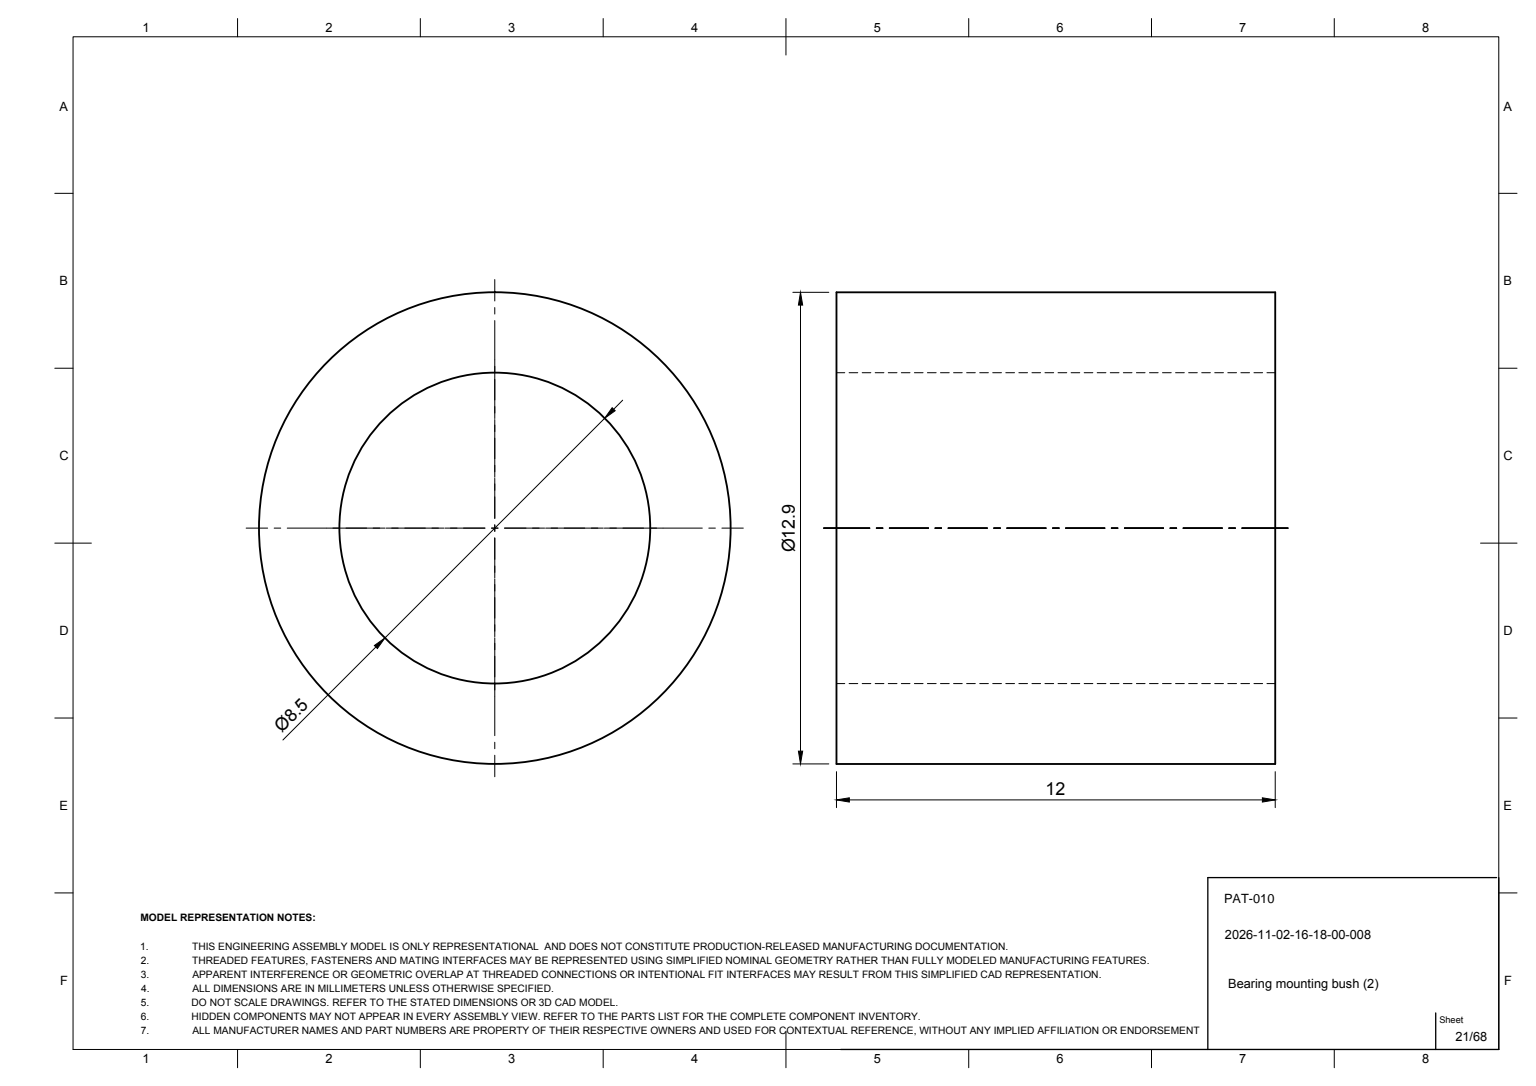
ISO-10303-21;
HEADER;
/* Generated by software containing ST-Developer
 * from STEP Tools, Inc. (www.steptools.com) 
 */

FILE_DESCRIPTION(
/* description */ ('Belt conveyor head drive unit'),
/* implementation_level */ '2;1');

FILE_NAME(
/* name */ 'Bearing mounting bush (2).step',
/* time_stamp */ '2026-10-28T03:26:19-07:00',
/* author */ (''),
/* organization */ (''),
/* preprocessor_version */ 'ST-DEVELOPER v20.2',
/* originating_system */ 'Autodesk Translation Framework v15.17.0.0',
/* authorisation */ '');

FILE_SCHEMA (('AUTOMOTIVE_DESIGN { 1 0 10303 214 3 1 1 }'));
ENDSEC;

DATA;
#10=MECHANICAL_DESIGN_GEOMETRIC_PRESENTATION_REPRESENTATION('',(#867),#27069);
#729=SHAPE_REPRESENTATION_RELATIONSHIP('SRR','None',#27373,#798);
#798=ADVANCED_BREP_SHAPE_REPRESENTATION('',(#952),#27015);
#867=STYLED_ITEM('',(#27797),#952);
#952=MANIFOLD_SOLID_BREP('Body1',#13732);
#1125=FACE_BOUND('',#2799,.T.);
#1126=FACE_BOUND('',#2801,.T.);
#1401=PLANE('',#15105);
#1402=PLANE('',#15106);
#1883=FACE_OUTER_BOUND('',#2796,.T.);
#1884=FACE_OUTER_BOUND('',#2797,.T.);
#1885=FACE_OUTER_BOUND('',#2798,.T.);
#1886=FACE_OUTER_BOUND('',#2800,.T.);
#2796=EDGE_LOOP('',(#10056,#10057,#10058,#10059));
#2797=EDGE_LOOP('',(#10060,#10061,#10062,#10063));
#2798=EDGE_LOOP('',(#10064));
#2799=EDGE_LOOP('',(#10065));
#2800=EDGE_LOOP('',(#10066));
#2801=EDGE_LOOP('',(#10067));
#3783=LINE('',#22162,#4575);
#3784=LINE('',#22168,#4576);
#4575=VECTOR('',#17797,0.425);
#4576=VECTOR('',#17804,0.645);
#5346=CIRCLE('',#15100,0.425);
#5347=CIRCLE('',#15101,0.425);
#5348=CIRCLE('',#15103,0.645);
#5349=CIRCLE('',#15104,0.645);
#6319=VERTEX_POINT('',#22159);
#6320=VERTEX_POINT('',#22161);
#6321=VERTEX_POINT('',#22165);
#6322=VERTEX_POINT('',#22167);
#7720=EDGE_CURVE('',#6319,#6319,#5346,.T.);
#7721=EDGE_CURVE('',#6319,#6320,#3783,.T.);
#7722=EDGE_CURVE('',#6320,#6320,#5347,.T.);
#7723=EDGE_CURVE('',#6321,#6321,#5348,.T.);
#7724=EDGE_CURVE('',#6321,#6322,#3784,.T.);
#7725=EDGE_CURVE('',#6322,#6322,#5349,.T.);
#10056=ORIENTED_EDGE('',*,*,#7720,.F.);
#10057=ORIENTED_EDGE('',*,*,#7721,.T.);
#10058=ORIENTED_EDGE('',*,*,#7722,.T.);
#10059=ORIENTED_EDGE('',*,*,#7721,.F.);
#10060=ORIENTED_EDGE('',*,*,#7723,.F.);
#10061=ORIENTED_EDGE('',*,*,#7724,.T.);
#10062=ORIENTED_EDGE('',*,*,#7725,.T.);
#10063=ORIENTED_EDGE('',*,*,#7724,.F.);
#10064=ORIENTED_EDGE('',*,*,#7723,.T.);
#10065=ORIENTED_EDGE('',*,*,#7720,.T.);
#10066=ORIENTED_EDGE('',*,*,#7725,.F.);
#10067=ORIENTED_EDGE('',*,*,#7722,.F.);
#12658=CYLINDRICAL_SURFACE('',#15099,0.425);
#12659=CYLINDRICAL_SURFACE('',#15102,0.645);
#13162=ADVANCED_FACE('',(#1883),#12658,.F.);
#13163=ADVANCED_FACE('',(#1884),#12659,.T.);
#13164=ADVANCED_FACE('',(#1885,#1125),#1401,.T.);
#13165=ADVANCED_FACE('',(#1886,#1126),#1402,.F.);
#13732=CLOSED_SHELL('',(#13162,#13163,#13164,#13165));
#15098=AXIS2_PLACEMENT_3D('',#22157,#17791,#17792);
#15099=AXIS2_PLACEMENT_3D('',#22158,#17793,#17794);
#15100=AXIS2_PLACEMENT_3D('',#22160,#17795,#17796);
#15101=AXIS2_PLACEMENT_3D('',#22163,#17798,#17799);
#15102=AXIS2_PLACEMENT_3D('',#22164,#17800,#17801);
#15103=AXIS2_PLACEMENT_3D('',#22166,#17802,#17803);
#15104=AXIS2_PLACEMENT_3D('',#22169,#17805,#17806);
#15105=AXIS2_PLACEMENT_3D('',#22170,#17807,#17808);
#15106=AXIS2_PLACEMENT_3D('',#22171,#17809,#17810);
#17791=DIRECTION('axis',(0.,0.,1.));
#17792=DIRECTION('refdir',(1.,0.,0.));
#17793=DIRECTION('center_axis',(0.,0.,1.));
#17794=DIRECTION('ref_axis',(1.,0.,0.));
#17795=DIRECTION('center_axis',(0.,0.,-1.));
#17796=DIRECTION('ref_axis',(1.,0.,0.));
#17797=DIRECTION('',(0.,0.,-1.));
#17798=DIRECTION('center_axis',(0.,0.,-1.));
#17799=DIRECTION('ref_axis',(1.,0.,0.));
#17800=DIRECTION('center_axis',(0.,0.,1.));
#17801=DIRECTION('ref_axis',(1.,0.,0.));
#17802=DIRECTION('center_axis',(0.,0.,1.));
#17803=DIRECTION('ref_axis',(1.,0.,0.));
#17804=DIRECTION('',(0.,0.,-1.));
#17805=DIRECTION('center_axis',(0.,0.,1.));
#17806=DIRECTION('ref_axis',(1.,0.,0.));
#17807=DIRECTION('center_axis',(0.,0.,1.));
#17808=DIRECTION('ref_axis',(1.,0.,0.));
#17809=DIRECTION('center_axis',(0.,0.,1.));
#17810=DIRECTION('ref_axis',(1.,0.,0.));
#22157=CARTESIAN_POINT('',(0.,0.,0.));
#22158=CARTESIAN_POINT('Origin',(2.22091003018116,40.,3.67));
#22159=CARTESIAN_POINT('',(1.79591003018116,40.,4.87));
#22160=CARTESIAN_POINT('Origin',(2.22091003018116,40.,4.87));
#22161=CARTESIAN_POINT('',(1.79591003018116,40.,3.67));
#22162=CARTESIAN_POINT('',(1.79591003018116,40.,3.67));
#22163=CARTESIAN_POINT('Origin',(2.22091003018116,40.,3.67));
#22164=CARTESIAN_POINT('Origin',(2.22091003018116,40.,3.67));
#22165=CARTESIAN_POINT('',(1.57591003018116,40.,4.87));
#22166=CARTESIAN_POINT('Origin',(2.22091003018116,40.,4.87));
#22167=CARTESIAN_POINT('',(1.57591003018116,40.,3.67));
#22168=CARTESIAN_POINT('',(1.57591003018116,40.,3.67));
#22169=CARTESIAN_POINT('Origin',(2.22091003018116,40.,3.67));
#22170=CARTESIAN_POINT('Origin',(2.22091003018116,40.,4.87));
#22171=CARTESIAN_POINT('Origin',(2.22091003018116,40.,3.67));
#26938=UNCERTAINTY_MEASURE_WITH_UNIT(LENGTH_MEASURE(0.001),#27070,
'DISTANCE_ACCURACY_VALUE',
'Maximum model space distance between geometric entities at asserted c
onnectivities');
#26992=UNCERTAINTY_MEASURE_WITH_UNIT(LENGTH_MEASURE(0.001),#27070,
'DISTANCE_ACCURACY_VALUE',
'Maximum model space distance between geometric entities at asserted c
onnectivities');
#27015=(
GEOMETRIC_REPRESENTATION_CONTEXT(3)
GLOBAL_UNCERTAINTY_ASSIGNED_CONTEXT((#26938))
GLOBAL_UNIT_ASSIGNED_CONTEXT((#27070,#27072,#27073))
REPRESENTATION_CONTEXT('','3D')
);
#27069=(
GEOMETRIC_REPRESENTATION_CONTEXT(3)
GLOBAL_UNCERTAINTY_ASSIGNED_CONTEXT((#26992))
GLOBAL_UNIT_ASSIGNED_CONTEXT((#27070,#27072,#27073))
REPRESENTATION_CONTEXT('','3D')
);
#27070=(
LENGTH_UNIT()
NAMED_UNIT(*)
SI_UNIT(.CENTI.,.METRE.)
);
#27072=(
NAMED_UNIT(*)
PLANE_ANGLE_UNIT()
SI_UNIT($,.RADIAN.)
);
#27073=(
NAMED_UNIT(*)
SI_UNIT($,.STERADIAN.)
SOLID_ANGLE_UNIT()
);
#27096=SHAPE_DEFINITION_REPRESENTATION(#27172,#27373);
#27172=PRODUCT_DEFINITION_SHAPE('',$,#27450);
#27373=SHAPE_REPRESENTATION('',(#15098),#27015);
#27427=PRODUCT_DEFINITION_CONTEXT('part definition',#27657,'design');
#27450=PRODUCT_DEFINITION('Bearing mounting bush (2)',
'Bearing mounting bush (2)',#27526,#27427);
#27526=PRODUCT_DEFINITION_FORMATION('',$,#27681);
#27657=APPLICATION_CONTEXT(
'Core Data for Automotive Mechanical Design Process');
#27658=PRODUCT_CONTEXT('part definition',#27657,'mechanical');
#27681=PRODUCT('Bearing mounting bush (2)','Bearing mounting bush (2)',
'Bearing mounting bush (2)',(#27658));
#27791=COLOUR_RGB('Grey',0.48,0.52,0.57);
#27792=FILL_AREA_STYLE_COLOUR('',#27791);
#27793=FILL_AREA_STYLE('',(#27792));
#27794=SURFACE_STYLE_FILL_AREA(#27793);
#27795=SURFACE_SIDE_STYLE('',(#27794));
#27796=SURFACE_STYLE_USAGE(.BOTH.,#27795);
#27797=PRESENTATION_STYLE_ASSIGNMENT((#27796));
ENDSEC;
END-ISO-10303-21;
